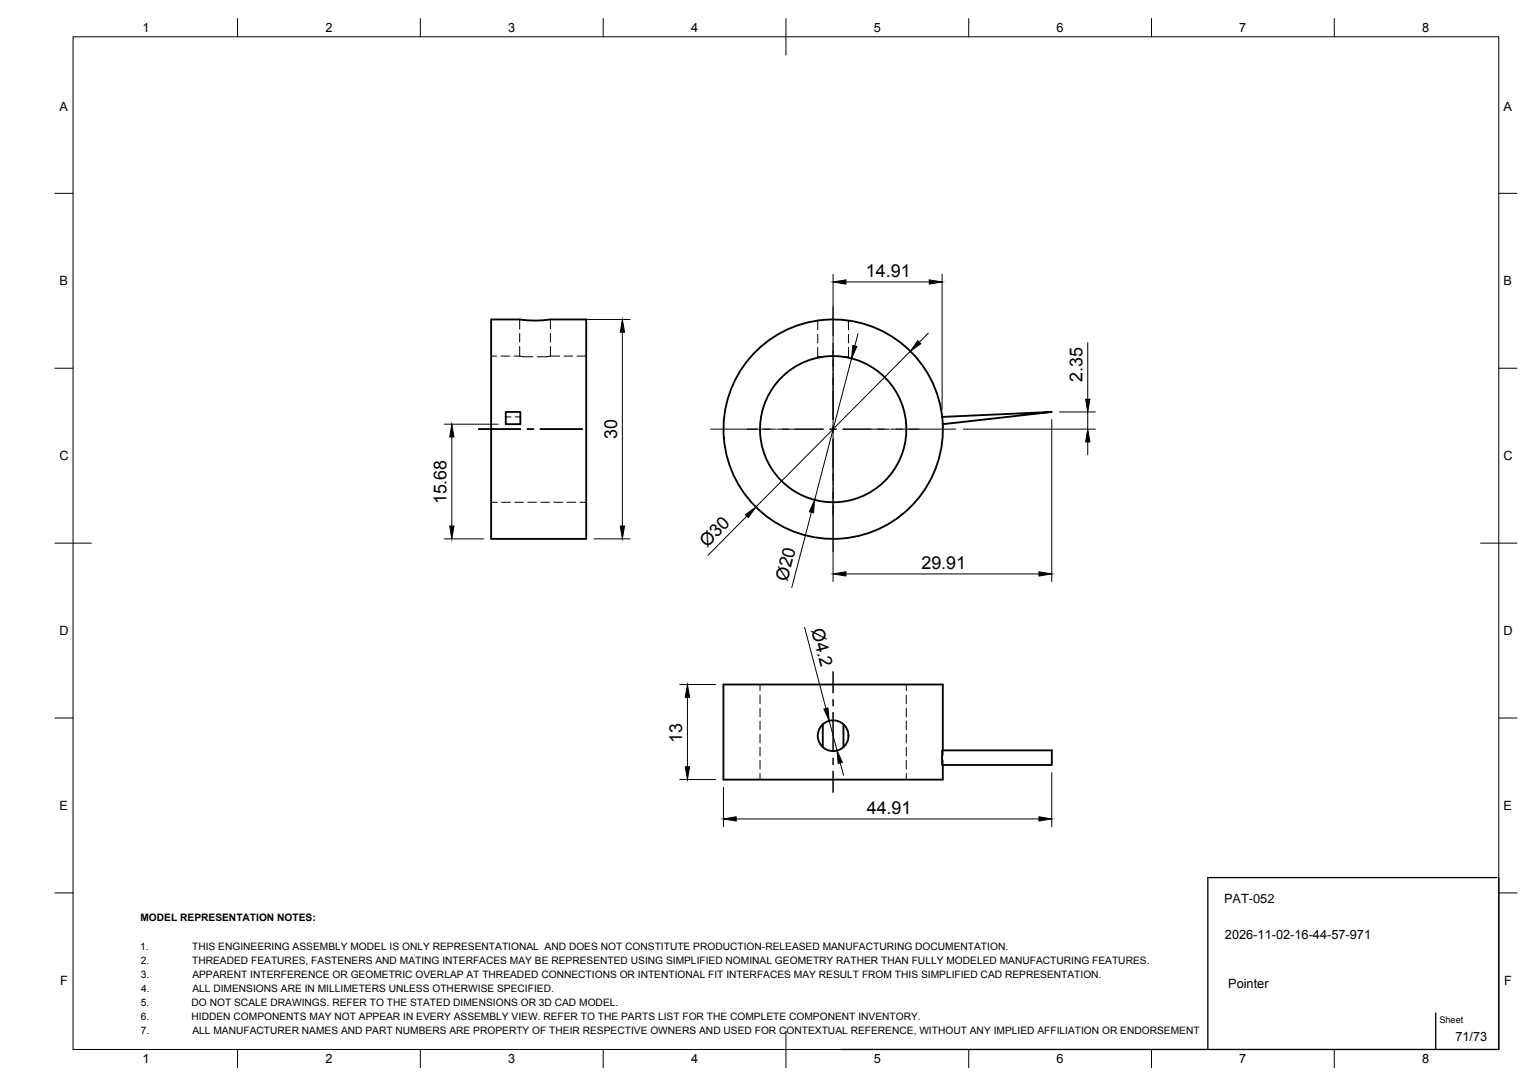
ISO-10303-21;
HEADER;
/* Generated by software containing ST-Developer
 * from STEP Tools, Inc. (www.steptools.com) 
 */

FILE_DESCRIPTION(
/* description */ ('Hand-crank gear train demonstrator'),
/* implementation_level */ '2;1');

FILE_NAME(
/* name */ 'Pointer.step',
/* time_stamp */ '2026-10-28T03:22:13-07:00',
/* author */ (''),
/* organization */ (''),
/* preprocessor_version */ 'ST-DEVELOPER v20.2',
/* originating_system */ 'Autodesk Translation Framework v15.17.0.0',
/* authorisation */ '');

FILE_SCHEMA (('AUTOMOTIVE_DESIGN { 1 0 10303 214 3 1 1 }'));
ENDSEC;

DATA;
#10=MECHANICAL_DESIGN_GEOMETRIC_PRESENTATION_REPRESENTATION('',(#1261),#62758);
#907=B_SPLINE_CURVE_WITH_KNOTS('',3,(#38641,#38642,#38643,#38644,#38645,
#38646,#38647,#38648,#38649,#38650),.UNSPECIFIED.,.F.,.F.,(4,2,2,2,4),(0.803821788694094,
0.872950991853624,0.952307212900975,1.03166343394833,1.10079263710785),
 .UNSPECIFIED.);
#908=B_SPLINE_CURVE_WITH_KNOTS('',3,(#38656,#38657,#38658,#38659,#38660,
#38661,#38662,#38663,#38664,#38665,#38666,#38667,#38668,#38669,#38670,#38671,
#38672,#38673),.UNSPECIFIED.,.F.,.F.,(4,2,2,2,2,2,2,2,4),(0.,0.0792165807733629,
0.158433161546726,0.237648697074571,0.316864232602417,0.396079768130262,
0.475295303658107,0.55451188443147,0.633728465204833),.UNSPECIFIED.);
#909=B_SPLINE_CURVE_WITH_KNOTS('',3,(#38674,#38675,#38676,#38677,#38678,
#38679,#38680,#38681,#38682,#38683,#38684,#38685,#38686,#38687,#38688,#38689,
#38690,#38691),.UNSPECIFIED.,.F.,.F.,(4,2,2,2,2,2,2,2,4),(0.633728465204833,
0.712945045978196,0.792161626751559,0.871377162279404,0.95059269780725,
1.0298082333351,1.10902376886294,1.1882403496363,1.26745693040967),
 .UNSPECIFIED.);
#910=B_SPLINE_CURVE_WITH_KNOTS('',3,(#38694,#38695,#38696,#38697,#38698,
#38699,#38700,#38701,#38702,#38703),.UNSPECIFIED.,.F.,.F.,(4,2,2,2,4),(0.168950313426782,
0.238079516586308,0.317435737633658,0.396791958681009,0.465921161840539),
 .UNSPECIFIED.);
#1118=SHAPE_REPRESENTATION_RELATIONSHIP('SRR','None',#63096,#1182);
#1182=ADVANCED_BREP_SHAPE_REPRESENTATION('',(#1336),#62750);
#1261=STYLED_ITEM('',(#63455),#1336);
#1336=MANIFOLD_SOLID_BREP('Body1',#16445);
#1619=FACE_BOUND('',#4054,.T.);
#1620=FACE_BOUND('',#4056,.T.);
#1621=FACE_BOUND('',#4057,.T.);
#1622=FACE_BOUND('',#4059,.T.);
#1623=FACE_BOUND('',#4061,.T.);
#2035=PLANE('',#18453);
#2036=PLANE('',#18458);
#2037=PLANE('',#18459);
#2038=PLANE('',#18460);
#2039=PLANE('',#18462);
#2040=PLANE('',#18464);
#2041=PLANE('',#18471);
#2042=PLANE('',#18472);
#2833=FACE_OUTER_BOUND('',#4046,.T.);
#2834=FACE_OUTER_BOUND('',#4047,.T.);
#2835=FACE_OUTER_BOUND('',#4048,.T.);
#2836=FACE_OUTER_BOUND('',#4049,.T.);
#2837=FACE_OUTER_BOUND('',#4050,.T.);
#2838=FACE_OUTER_BOUND('',#4051,.T.);
#2839=FACE_OUTER_BOUND('',#4052,.T.);
#2840=FACE_OUTER_BOUND('',#4053,.T.);
#2841=FACE_OUTER_BOUND('',#4055,.T.);
#2842=FACE_OUTER_BOUND('',#4058,.T.);
#2843=FACE_OUTER_BOUND('',#4060,.T.);
#4046=EDGE_LOOP('',(#13941,#13942));
#4047=EDGE_LOOP('',(#13943,#13944,#13945,#13946,#13947,#13948,#13949,#13950,
#13951));
#4048=EDGE_LOOP('',(#13952,#13953,#13954));
#4049=EDGE_LOOP('',(#13955,#13956,#13957,#13958));
#4050=EDGE_LOOP('',(#13959,#13960,#13961));
#4051=EDGE_LOOP('',(#13962,#13963,#13964));
#4052=EDGE_LOOP('',(#13965,#13966,#13967,#13968));
#4053=EDGE_LOOP('',(#13969,#13970,#13971,#13972));
#4054=EDGE_LOOP('',(#13973,#13974,#13975,#13976));
#4055=EDGE_LOOP('',(#13977,#13978,#13979,#13980));
#4056=EDGE_LOOP('',(#13981,#13982));
#4057=EDGE_LOOP('',(#13983,#13984,#13985,#13986));
#4058=EDGE_LOOP('',(#13987));
#4059=EDGE_LOOP('',(#13988));
#4060=EDGE_LOOP('',(#13989));
#4061=EDGE_LOOP('',(#13990));
#5162=LINE('',#38637,#6294);
#5163=LINE('',#38654,#6295);
#5164=LINE('',#38705,#6296);
#5165=LINE('',#38709,#6297);
#5166=LINE('',#38711,#6298);
#5167=LINE('',#38713,#6299);
#5168=LINE('',#38714,#6300);
#5169=LINE('',#38718,#6301);
#5170=LINE('',#38722,#6302);
#5171=LINE('',#38724,#6303);
#5172=LINE('',#38729,#6304);
#5173=LINE('',#38735,#6305);
#6294=VECTOR('',#22299,1.);
#6295=VECTOR('',#22306,0.210000000000001);
#6296=VECTOR('',#22311,1.);
#6297=VECTOR('',#22314,1.);
#6298=VECTOR('',#22315,1.);
#6299=VECTOR('',#22316,1.);
#6300=VECTOR('',#22317,1.);
#6301=VECTOR('',#22322,1.);
#6302=VECTOR('',#22327,1.);
#6303=VECTOR('',#22330,1.);
#6304=VECTOR('',#22335,1.);
#6305=VECTOR('',#22342,1.5);
#7099=CIRCLE('',#18454,0.210000000000001);
#7100=CIRCLE('',#18456,0.210000000000001);
#7101=CIRCLE('',#18457,0.210000000000001);
#7102=CIRCLE('',#18461,1.5);
#7103=CIRCLE('',#18463,1.5);
#7104=CIRCLE('',#18466,1.);
#7105=CIRCLE('',#18467,1.);
#7106=CIRCLE('',#18469,1.5);
#7107=CIRCLE('',#18470,1.5);
#8262=VERTEX_POINT('',#38635);
#8263=VERTEX_POINT('',#38636);
#8264=VERTEX_POINT('',#38640);
#8265=VERTEX_POINT('',#38651);
#8266=VERTEX_POINT('',#38653);
#8267=VERTEX_POINT('',#38655);
#8268=VERTEX_POINT('',#38692);
#8269=VERTEX_POINT('',#38707);
#8270=VERTEX_POINT('',#38708);
#8271=VERTEX_POINT('',#38710);
#8272=VERTEX_POINT('',#38712);
#8273=VERTEX_POINT('',#38716);
#8274=VERTEX_POINT('',#38720);
#8275=VERTEX_POINT('',#38726);
#8276=VERTEX_POINT('',#38728);
#8277=VERTEX_POINT('',#38732);
#8278=VERTEX_POINT('',#38734);
#10222=EDGE_CURVE('',#8262,#8263,#5162,.T.);
#10223=EDGE_CURVE('',#8262,#8263,#7099,.T.);
#10224=EDGE_CURVE('',#8264,#8262,#907,.T.);
#10225=EDGE_CURVE('',#8265,#8264,#7100,.T.);
#10226=EDGE_CURVE('',#8265,#8266,#5163,.T.);
#10227=EDGE_CURVE('',#8267,#8266,#908,.T.);
#10228=EDGE_CURVE('',#8266,#8267,#909,.T.);
#10229=EDGE_CURVE('',#8268,#8265,#7101,.T.);
#10230=EDGE_CURVE('',#8263,#8268,#910,.T.);
#10231=EDGE_CURVE('',#8268,#8264,#5164,.T.);
#10232=EDGE_CURVE('',#8269,#8270,#5165,.T.);
#10233=EDGE_CURVE('',#8269,#8271,#5166,.T.);
#10234=EDGE_CURVE('',#8271,#8272,#5167,.T.);
#10235=EDGE_CURVE('',#8270,#8272,#5168,.T.);
#10236=EDGE_CURVE('',#8273,#8269,#7102,.T.);
#10237=EDGE_CURVE('',#8271,#8273,#5169,.T.);
#10238=EDGE_CURVE('',#8270,#8274,#7103,.T.);
#10239=EDGE_CURVE('',#8272,#8274,#5170,.T.);
#10240=EDGE_CURVE('',#8274,#8273,#5171,.T.);
#10241=EDGE_CURVE('',#8275,#8275,#7104,.T.);
#10242=EDGE_CURVE('',#8275,#8276,#5172,.T.);
#10243=EDGE_CURVE('',#8276,#8276,#7105,.T.);
#10244=EDGE_CURVE('',#8277,#8277,#7106,.T.);
#10245=EDGE_CURVE('',#8277,#8278,#5173,.T.);
#10246=EDGE_CURVE('',#8278,#8278,#7107,.T.);
#13941=ORIENTED_EDGE('',*,*,#10222,.F.);
#13942=ORIENTED_EDGE('',*,*,#10223,.T.);
#13943=ORIENTED_EDGE('',*,*,#10224,.F.);
#13944=ORIENTED_EDGE('',*,*,#10225,.F.);
#13945=ORIENTED_EDGE('',*,*,#10226,.T.);
#13946=ORIENTED_EDGE('',*,*,#10227,.F.);
#13947=ORIENTED_EDGE('',*,*,#10228,.F.);
#13948=ORIENTED_EDGE('',*,*,#10226,.F.);
#13949=ORIENTED_EDGE('',*,*,#10229,.F.);
#13950=ORIENTED_EDGE('',*,*,#10230,.F.);
#13951=ORIENTED_EDGE('',*,*,#10223,.F.);
#13952=ORIENTED_EDGE('',*,*,#10231,.F.);
#13953=ORIENTED_EDGE('',*,*,#10229,.T.);
#13954=ORIENTED_EDGE('',*,*,#10225,.T.);
#13955=ORIENTED_EDGE('',*,*,#10232,.F.);
#13956=ORIENTED_EDGE('',*,*,#10233,.T.);
#13957=ORIENTED_EDGE('',*,*,#10234,.T.);
#13958=ORIENTED_EDGE('',*,*,#10235,.F.);
#13959=ORIENTED_EDGE('',*,*,#10236,.F.);
#13960=ORIENTED_EDGE('',*,*,#10237,.F.);
#13961=ORIENTED_EDGE('',*,*,#10233,.F.);
#13962=ORIENTED_EDGE('',*,*,#10238,.F.);
#13963=ORIENTED_EDGE('',*,*,#10235,.T.);
#13964=ORIENTED_EDGE('',*,*,#10239,.T.);
#13965=ORIENTED_EDGE('',*,*,#10240,.F.);
#13966=ORIENTED_EDGE('',*,*,#10239,.F.);
#13967=ORIENTED_EDGE('',*,*,#10234,.F.);
#13968=ORIENTED_EDGE('',*,*,#10237,.T.);
#13969=ORIENTED_EDGE('',*,*,#10241,.F.);
#13970=ORIENTED_EDGE('',*,*,#10242,.T.);
#13971=ORIENTED_EDGE('',*,*,#10243,.T.);
#13972=ORIENTED_EDGE('',*,*,#10242,.F.);
#13973=ORIENTED_EDGE('',*,*,#10230,.T.);
#13974=ORIENTED_EDGE('',*,*,#10231,.T.);
#13975=ORIENTED_EDGE('',*,*,#10224,.T.);
#13976=ORIENTED_EDGE('',*,*,#10222,.T.);
#13977=ORIENTED_EDGE('',*,*,#10244,.F.);
#13978=ORIENTED_EDGE('',*,*,#10245,.T.);
#13979=ORIENTED_EDGE('',*,*,#10246,.T.);
#13980=ORIENTED_EDGE('',*,*,#10245,.F.);
#13981=ORIENTED_EDGE('',*,*,#10227,.T.);
#13982=ORIENTED_EDGE('',*,*,#10228,.T.);
#13983=ORIENTED_EDGE('',*,*,#10240,.T.);
#13984=ORIENTED_EDGE('',*,*,#10236,.T.);
#13985=ORIENTED_EDGE('',*,*,#10232,.T.);
#13986=ORIENTED_EDGE('',*,*,#10238,.T.);
#13987=ORIENTED_EDGE('',*,*,#10244,.T.);
#13988=ORIENTED_EDGE('',*,*,#10241,.T.);
#13989=ORIENTED_EDGE('',*,*,#10246,.F.);
#13990=ORIENTED_EDGE('',*,*,#10243,.F.);
#15381=CYLINDRICAL_SURFACE('',#18455,0.210000000000001);
#15382=CYLINDRICAL_SURFACE('',#18465,1.);
#15383=CYLINDRICAL_SURFACE('',#18468,1.5);
#16143=ADVANCED_FACE('',(#2833),#2035,.T.);
#16144=ADVANCED_FACE('',(#2834),#15381,.F.);
#16145=ADVANCED_FACE('',(#2835),#2036,.T.);
#16146=ADVANCED_FACE('',(#2836),#2037,.T.);
#16147=ADVANCED_FACE('',(#2837),#2038,.F.);
#16148=ADVANCED_FACE('',(#2838),#2039,.T.);
#16149=ADVANCED_FACE('',(#2839),#2040,.T.);
#16150=ADVANCED_FACE('',(#2840,#1619),#15382,.F.);
#16151=ADVANCED_FACE('',(#2841,#1620,#1621),#15383,.T.);
#16152=ADVANCED_FACE('',(#2842,#1622),#2041,.T.);
#16153=ADVANCED_FACE('',(#2843,#1623),#2042,.F.);
#16445=CLOSED_SHELL('',(#16143,#16144,#16145,#16146,#16147,#16148,#16149,
#16150,#16151,#16152,#16153));
#18452=AXIS2_PLACEMENT_3D('',#38633,#22295,#22296);
#18453=AXIS2_PLACEMENT_3D('',#38634,#22297,#22298);
#18454=AXIS2_PLACEMENT_3D('',#38638,#22300,#22301);
#18455=AXIS2_PLACEMENT_3D('',#38639,#22302,#22303);
#18456=AXIS2_PLACEMENT_3D('',#38652,#22304,#22305);
#18457=AXIS2_PLACEMENT_3D('',#38693,#22307,#22308);
#18458=AXIS2_PLACEMENT_3D('',#38704,#22309,#22310);
#18459=AXIS2_PLACEMENT_3D('',#38706,#22312,#22313);
#18460=AXIS2_PLACEMENT_3D('',#38715,#22318,#22319);
#18461=AXIS2_PLACEMENT_3D('',#38717,#22320,#22321);
#18462=AXIS2_PLACEMENT_3D('',#38719,#22323,#22324);
#18463=AXIS2_PLACEMENT_3D('',#38721,#22325,#22326);
#18464=AXIS2_PLACEMENT_3D('',#38723,#22328,#22329);
#18465=AXIS2_PLACEMENT_3D('',#38725,#22331,#22332);
#18466=AXIS2_PLACEMENT_3D('',#38727,#22333,#22334);
#18467=AXIS2_PLACEMENT_3D('',#38730,#22336,#22337);
#18468=AXIS2_PLACEMENT_3D('',#38731,#22338,#22339);
#18469=AXIS2_PLACEMENT_3D('',#38733,#22340,#22341);
#18470=AXIS2_PLACEMENT_3D('',#38736,#22343,#22344);
#18471=AXIS2_PLACEMENT_3D('',#38737,#22345,#22346);
#18472=AXIS2_PLACEMENT_3D('',#38738,#22347,#22348);
#22295=DIRECTION('axis',(0.,0.,1.));
#22296=DIRECTION('refdir',(1.,0.,0.));
#22297=DIRECTION('center_axis',(0.,0.,1.));
#22298=DIRECTION('ref_axis',(1.,0.,0.));
#22299=DIRECTION('',(0.,1.,0.));
#22300=DIRECTION('center_axis',(0.,0.,1.));
#22301=DIRECTION('ref_axis',(1.,0.,0.));
#22302=DIRECTION('center_axis',(0.,0.,1.));
#22303=DIRECTION('ref_axis',(1.,0.,0.));
#22304=DIRECTION('center_axis',(0.,0.,1.));
#22305=DIRECTION('ref_axis',(1.,0.,0.));
#22306=DIRECTION('',(0.,0.,1.));
#22307=DIRECTION('center_axis',(0.,0.,1.));
#22308=DIRECTION('ref_axis',(1.,0.,0.));
#22309=DIRECTION('center_axis',(0.,0.,1.));
#22310=DIRECTION('ref_axis',(1.,0.,0.));
#22311=DIRECTION('',(0.,-1.,0.));
#22312=DIRECTION('center_axis',(-0.045218998239459,0.,0.998977097934793));
#22313=DIRECTION('ref_axis',(0.998977097934793,0.,0.045218998239459));
#22314=DIRECTION('',(0.,1.,0.));
#22315=DIRECTION('',(0.998977097934793,0.,0.045218998239459));
#22316=DIRECTION('',(0.,1.,0.));
#22317=DIRECTION('',(0.998977097934793,0.,0.045218998239459));
#22318=DIRECTION('center_axis',(0.,1.,0.));
#22319=DIRECTION('ref_axis',(1.,0.,0.));
#22320=DIRECTION('center_axis',(0.,-1.,0.));
#22321=DIRECTION('ref_axis',(1.,0.,0.));
#22322=DIRECTION('',(-0.993771205694266,0.,-0.111439628198257));
#22323=DIRECTION('center_axis',(0.,1.,0.));
#22324=DIRECTION('ref_axis',(0.,0.,1.));
#22325=DIRECTION('center_axis',(0.,1.,0.));
#22326=DIRECTION('ref_axis',(1.,0.,0.));
#22327=DIRECTION('',(-0.993771205694266,0.,-0.111439628198257));
#22328=DIRECTION('center_axis',(0.111439628198257,0.,-0.993771205694266));
#22329=DIRECTION('ref_axis',(-0.993771205694266,0.,-0.111439628198257));
#22330=DIRECTION('',(0.,-1.,0.));
#22331=DIRECTION('center_axis',(0.,1.,0.));
#22332=DIRECTION('ref_axis',(1.,0.,0.));
#22333=DIRECTION('center_axis',(0.,-1.,0.));
#22334=DIRECTION('ref_axis',(1.,0.,0.));
#22335=DIRECTION('',(0.,-1.,0.));
#22336=DIRECTION('center_axis',(0.,-1.,0.));
#22337=DIRECTION('ref_axis',(1.,0.,0.));
#22338=DIRECTION('center_axis',(0.,1.,0.));
#22339=DIRECTION('ref_axis',(1.,0.,0.));
#22340=DIRECTION('center_axis',(0.,1.,0.));
#22341=DIRECTION('ref_axis',(1.,0.,0.));
#22342=DIRECTION('',(0.,-1.,0.));
#22343=DIRECTION('center_axis',(0.,1.,0.));
#22344=DIRECTION('ref_axis',(1.,0.,0.));
#22345=DIRECTION('center_axis',(0.,1.,0.));
#22346=DIRECTION('ref_axis',(1.,0.,0.));
#22347=DIRECTION('center_axis',(0.,1.,0.));
#22348=DIRECTION('ref_axis',(1.,0.,0.));
#38633=CARTESIAN_POINT('',(0.,0.,0.));
#38634=CARTESIAN_POINT('Origin',(18.,4.8,9.99));
#38635=CARTESIAN_POINT('',(18.1410673597966,4.64443650813894,9.99));
#38636=CARTESIAN_POINT('',(18.1410673597966,4.95556349186105,9.99));
#38637=CARTESIAN_POINT('',(18.1410673597966,4.2,9.99));
#38638=CARTESIAN_POINT('Origin',(18.,4.8,9.99));
#38639=CARTESIAN_POINT('Origin',(18.,4.8,9.99));
#38640=CARTESIAN_POINT('',(17.8589326402034,4.64443650813894,9.99));
#38641=CARTESIAN_POINT('Ctrl Pts',(17.8589326402034,4.64443650813895,9.99));
#38642=CARTESIAN_POINT('Ctrl Pts',(17.8761816433018,4.6287948476368,9.99245784982447));
#38643=CARTESIAN_POINT('Ctrl Pts',(17.8970013568903,4.61537595666898,9.99493819304946));
#38644=CARTESIAN_POINT('Ctrl Pts',(17.9453858856016,4.59530253627557,9.99884449237241));
#38645=CARTESIAN_POINT('Ctrl Pts',(17.9735479263176,4.59,10.));
#38646=CARTESIAN_POINT('Ctrl Pts',(18.0264520736824,4.59,10.));
#38647=CARTESIAN_POINT('Ctrl Pts',(18.0546141143984,4.59530253627557,9.99884449237241));
#38648=CARTESIAN_POINT('Ctrl Pts',(18.1029986431097,4.61537595666898,9.99493819304946));
#38649=CARTESIAN_POINT('Ctrl Pts',(18.1238183566982,4.62879484763679,9.99245784982447));
#38650=CARTESIAN_POINT('Ctrl Pts',(18.1410673597966,4.64443650813894,9.99));
#38651=CARTESIAN_POINT('',(17.79,4.8,9.99));
#38652=CARTESIAN_POINT('Origin',(18.,4.8,9.99));
#38653=CARTESIAN_POINT('',(17.79,4.8,10.4852272553384));
#38654=CARTESIAN_POINT('',(17.79,4.8,9.99));
#38655=CARTESIAN_POINT('',(18.21,4.8,10.4852272553384));
#38656=CARTESIAN_POINT('Ctrl Pts',(18.21,4.8,10.4852272553384));
#38657=CARTESIAN_POINT('Ctrl Pts',(18.21,4.77359447307555,10.4852272553384));
#38658=CARTESIAN_POINT('Ctrl Pts',(18.2047157372696,4.74545292590929,10.4860041595441));
#38659=CARTESIAN_POINT('Ctrl Pts',(18.1832737630363,4.69372373109487,10.4888007328232));
#38660=CARTESIAN_POINT('Ctrl Pts',(18.1671179239704,4.67013307587204,10.4907789715758));
#38661=CARTESIAN_POINT('Ctrl Pts',(18.1298671698874,4.63288232178902,10.4944848114133));
#38662=CARTESIAN_POINT('Ctrl Pts',(18.1062764083058,4.61672628999865,10.4964545565713));
#38663=CARTESIAN_POINT('Ctrl Pts',(18.0545468514059,4.59528417517378,10.4992316551565));
#38664=CARTESIAN_POINT('Ctrl Pts',(18.0264051785093,4.59,10.5));
#38665=CARTESIAN_POINT('Ctrl Pts',(17.9735948214907,4.59,10.5));
#38666=CARTESIAN_POINT('Ctrl Pts',(17.9454531485941,4.59528417517378,10.4992316551565));
#38667=CARTESIAN_POINT('Ctrl Pts',(17.8937235916942,4.61672628999865,10.4964545565713));
#38668=CARTESIAN_POINT('Ctrl Pts',(17.8701328301126,4.63288232178902,10.4944848114133));
#38669=CARTESIAN_POINT('Ctrl Pts',(17.8328820760296,4.67013307587204,10.4907789715758));
#38670=CARTESIAN_POINT('Ctrl Pts',(17.8167262369637,4.69372373109487,10.4888007328232));
#38671=CARTESIAN_POINT('Ctrl Pts',(17.7952842627304,4.74545292590929,10.4860041595441));
#38672=CARTESIAN_POINT('Ctrl Pts',(17.79,4.77359447307555,10.4852272553384));
#38673=CARTESIAN_POINT('Ctrl Pts',(17.79,4.8,10.4852272553384));
#38674=CARTESIAN_POINT('Ctrl Pts',(17.79,4.8,10.4852272553384));
#38675=CARTESIAN_POINT('Ctrl Pts',(17.79,4.82640552692445,10.4852272553384));
#38676=CARTESIAN_POINT('Ctrl Pts',(17.7952842627304,4.85454707409071,10.4860041595441));
#38677=CARTESIAN_POINT('Ctrl Pts',(17.8167262369637,4.90627626890513,10.4888007328232));
#38678=CARTESIAN_POINT('Ctrl Pts',(17.8328820760296,4.92986692412796,10.4907789715758));
#38679=CARTESIAN_POINT('Ctrl Pts',(17.8701328301126,4.96711767821098,10.4944848114133));
#38680=CARTESIAN_POINT('Ctrl Pts',(17.8937235916942,4.98327371000135,10.4964545565713));
#38681=CARTESIAN_POINT('Ctrl Pts',(17.9454531485941,5.00471582482622,10.4992316551565));
#38682=CARTESIAN_POINT('Ctrl Pts',(17.9735948214907,5.01,10.5));
#38683=CARTESIAN_POINT('Ctrl Pts',(18.0264051785093,5.01,10.5));
#38684=CARTESIAN_POINT('Ctrl Pts',(18.0545468514059,5.00471582482622,10.4992316551565));
#38685=CARTESIAN_POINT('Ctrl Pts',(18.1062764083058,4.98327371000135,10.4964545565713));
#38686=CARTESIAN_POINT('Ctrl Pts',(18.1298671698874,4.96711767821098,10.4944848114133));
#38687=CARTESIAN_POINT('Ctrl Pts',(18.1671179239704,4.92986692412796,10.4907789715758));
#38688=CARTESIAN_POINT('Ctrl Pts',(18.1832737630363,4.90627626890513,10.4888007328232));
#38689=CARTESIAN_POINT('Ctrl Pts',(18.2047157372696,4.85454707409071,10.4860041595441));
#38690=CARTESIAN_POINT('Ctrl Pts',(18.21,4.82640552692445,10.4852272553384));
#38691=CARTESIAN_POINT('Ctrl Pts',(18.21,4.8,10.4852272553384));
#38692=CARTESIAN_POINT('',(17.8589326402034,4.95556349186105,9.99));
#38693=CARTESIAN_POINT('Origin',(18.,4.8,9.99));
#38694=CARTESIAN_POINT('Ctrl Pts',(18.1410673597966,4.95556349186106,9.99));
#38695=CARTESIAN_POINT('Ctrl Pts',(18.1238183566982,4.97120515236321,9.99245784982447));
#38696=CARTESIAN_POINT('Ctrl Pts',(18.1029986431097,4.98462404333102,9.99493819304946));
#38697=CARTESIAN_POINT('Ctrl Pts',(18.0546141143984,5.00469746372443,9.99884449237241));
#38698=CARTESIAN_POINT('Ctrl Pts',(18.0264520736824,5.01,10.));
#38699=CARTESIAN_POINT('Ctrl Pts',(17.9735479263176,5.01,10.));
#38700=CARTESIAN_POINT('Ctrl Pts',(17.9453858856016,5.00469746372443,9.99884449237241));
#38701=CARTESIAN_POINT('Ctrl Pts',(17.8970013568903,4.98462404333102,9.99493819304946));
#38702=CARTESIAN_POINT('Ctrl Pts',(17.8761816433018,4.97120515236321,9.99245784982447));
#38703=CARTESIAN_POINT('Ctrl Pts',(17.8589326402034,4.95556349186105,9.99));
#38704=CARTESIAN_POINT('Origin',(18.,4.8,9.99));
#38705=CARTESIAN_POINT('',(17.8589326402034,4.2,9.99));
#38706=CARTESIAN_POINT('Origin',(18.,4.4,9.1));
#38707=CARTESIAN_POINT('',(19.4906215647723,4.4,9.16747343262672));
#38708=CARTESIAN_POINT('',(19.4906215647723,4.6,9.16747343262672));
#38709=CARTESIAN_POINT('',(19.4906215647723,4.2,9.16747343262672));
#38710=CARTESIAN_POINT('',(20.9907520011994,4.4,9.23537728718354));
#38711=CARTESIAN_POINT('',(18.,4.4,9.1));
#38712=CARTESIAN_POINT('',(20.9907520011994,4.6,9.23537728718354));
#38713=CARTESIAN_POINT('',(20.9907520011994,4.4,9.23537728718354));
#38714=CARTESIAN_POINT('',(18.,4.6,9.1));
#38715=CARTESIAN_POINT('Origin',(19.4953760005997,4.4,9.06768864359177));
#38716=CARTESIAN_POINT('',(19.4984563276619,4.4,9.06803406565731));
#38717=CARTESIAN_POINT('Origin',(18.,4.4,9.));
#38718=CARTESIAN_POINT('',(20.9907520011994,4.4,9.23537728718354));
#38719=CARTESIAN_POINT('Origin',(19.4953760005997,4.6,9.06768864359177));
#38720=CARTESIAN_POINT('',(19.4984563276619,4.6,9.06803406565731));
#38721=CARTESIAN_POINT('Origin',(18.,4.6,9.));
#38722=CARTESIAN_POINT('',(20.9907520011994,4.6,9.23537728718354));
#38723=CARTESIAN_POINT('Origin',(20.9907520011994,4.4,9.23537728718354));
#38724=CARTESIAN_POINT('',(19.4984563276619,4.2,9.06803406565731));
#38725=CARTESIAN_POINT('Origin',(18.,4.2,9.));
#38726=CARTESIAN_POINT('',(17.,5.5,9.));
#38727=CARTESIAN_POINT('Origin',(18.,5.5,9.));
#38728=CARTESIAN_POINT('',(17.,4.2,9.));
#38729=CARTESIAN_POINT('',(17.,4.2,9.));
#38730=CARTESIAN_POINT('Origin',(18.,4.2,9.));
#38731=CARTESIAN_POINT('Origin',(18.,4.2,9.));
#38732=CARTESIAN_POINT('',(16.5,5.5,9.));
#38733=CARTESIAN_POINT('Origin',(18.,5.5,9.));
#38734=CARTESIAN_POINT('',(16.5,4.2,9.));
#38735=CARTESIAN_POINT('',(16.5,4.2,9.));
#38736=CARTESIAN_POINT('Origin',(18.,4.2,9.));
#38737=CARTESIAN_POINT('Origin',(18.,5.5,9.));
#38738=CARTESIAN_POINT('Origin',(18.,4.2,9.));
#62676=UNCERTAINTY_MEASURE_WITH_UNIT(LENGTH_MEASURE(0.001),#62759,
'DISTANCE_ACCURACY_VALUE',
'Maximum model space distance between geometric entities at asserted c
onnectivities');
#62684=UNCERTAINTY_MEASURE_WITH_UNIT(LENGTH_MEASURE(0.001),#62759,
'DISTANCE_ACCURACY_VALUE',
'Maximum model space distance between geometric entities at asserted c
onnectivities');
#62750=(
GEOMETRIC_REPRESENTATION_CONTEXT(3)
GLOBAL_UNCERTAINTY_ASSIGNED_CONTEXT((#62676))
GLOBAL_UNIT_ASSIGNED_CONTEXT((#62759,#62761,#62762))
REPRESENTATION_CONTEXT('','3D')
);
#62758=(
GEOMETRIC_REPRESENTATION_CONTEXT(3)
GLOBAL_UNCERTAINTY_ASSIGNED_CONTEXT((#62684))
GLOBAL_UNIT_ASSIGNED_CONTEXT((#62759,#62761,#62762))
REPRESENTATION_CONTEXT('','3D')
);
#62759=(
LENGTH_UNIT()
NAMED_UNIT(*)
SI_UNIT(.CENTI.,.METRE.)
);
#62761=(
NAMED_UNIT(*)
PLANE_ANGLE_UNIT()
SI_UNIT($,.RADIAN.)
);
#62762=(
NAMED_UNIT(*)
SI_UNIT($,.STERADIAN.)
SOLID_ANGLE_UNIT()
);
#62828=SHAPE_DEFINITION_REPRESENTATION(#62911,#63096);
#62911=PRODUCT_DEFINITION_SHAPE('',$,#63170);
#63096=SHAPE_REPRESENTATION('',(#18452),#62750);
#63104=PRODUCT_DEFINITION_CONTEXT('part definition',#63325,'design');
#63170=PRODUCT_DEFINITION('Pointer','Pointer',#63243,#63104);
#63243=PRODUCT_DEFINITION_FORMATION('',$,#63392);
#63325=APPLICATION_CONTEXT(
'Core Data for Automotive Mechanical Design Process');
#63326=PRODUCT_CONTEXT('part definition',#63325,'mechanical');
#63392=PRODUCT('Pointer','Pointer','Pointer',(#63326));
#63449=COLOUR_RGB('Sky Blue',0.24,0.69,0.87);
#63450=FILL_AREA_STYLE_COLOUR('',#63449);
#63451=FILL_AREA_STYLE('',(#63450));
#63452=SURFACE_STYLE_FILL_AREA(#63451);
#63453=SURFACE_SIDE_STYLE('',(#63452));
#63454=SURFACE_STYLE_USAGE(.BOTH.,#63453);
#63455=PRESENTATION_STYLE_ASSIGNMENT((#63454));
ENDSEC;
END-ISO-10303-21;
